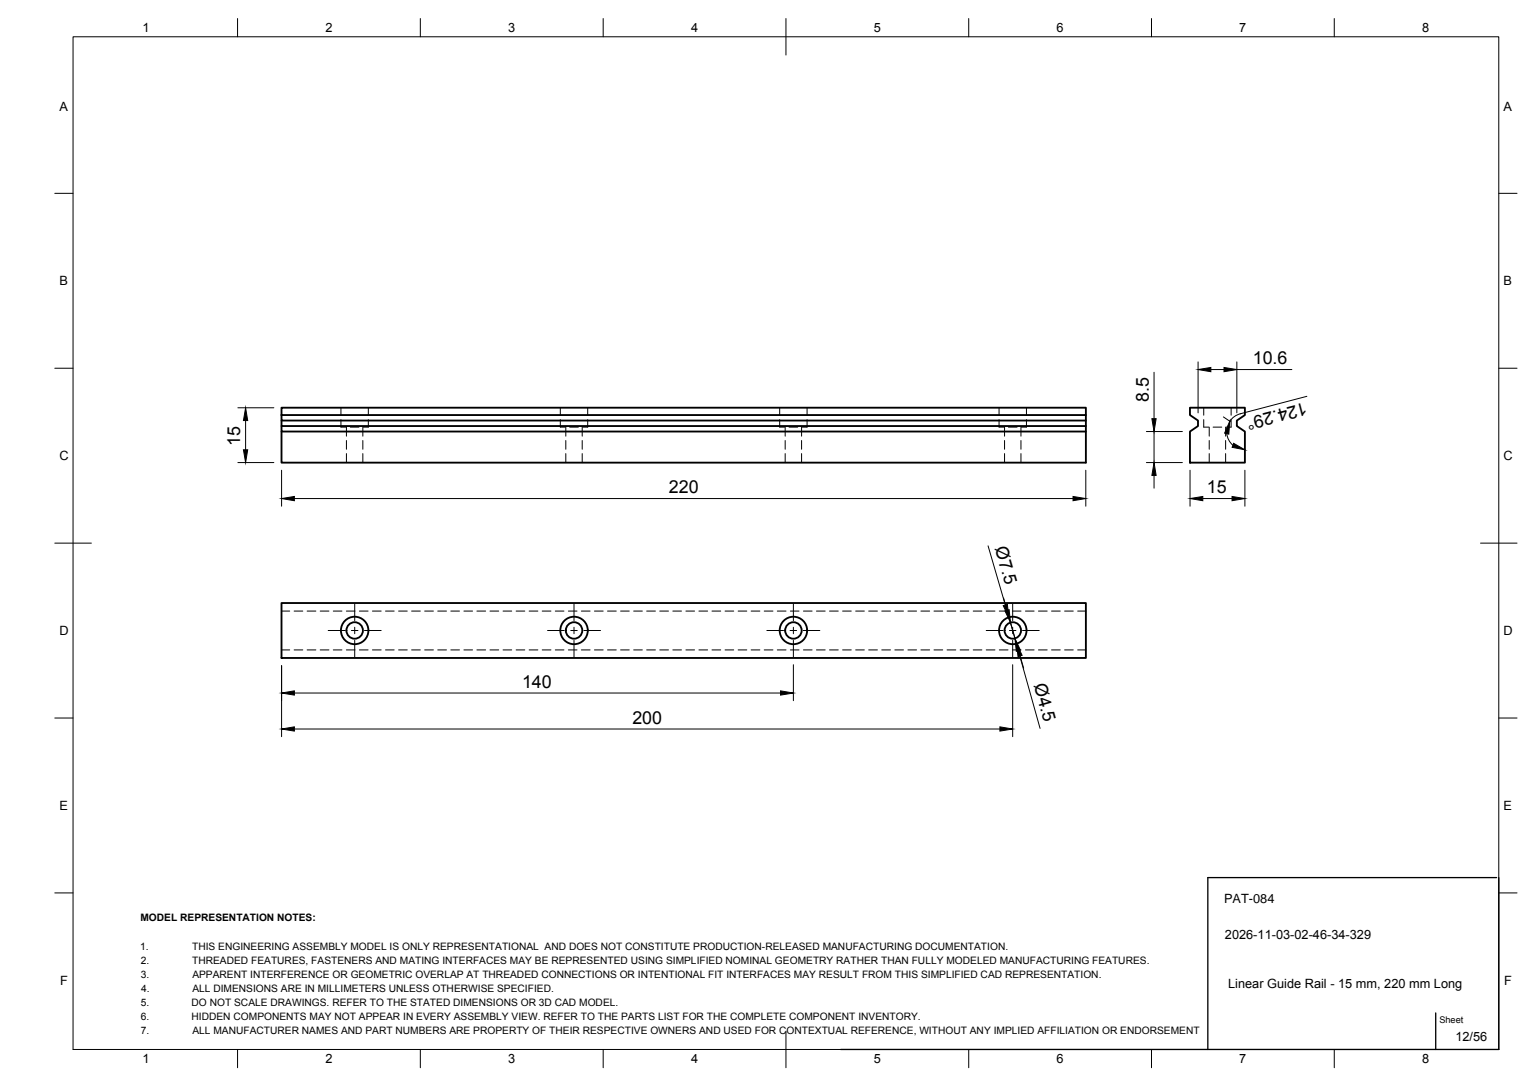
ISO-10303-21;
HEADER;
/* Generated by software containing ST-Developer
 * from STEP Tools, Inc. (www.steptools.com) 
 */

FILE_DESCRIPTION(
/* description */ ('Quick-return (Whitworth) mechanism'),
/* implementation_level */ '2;1');

FILE_NAME(
/* name */ 'Linear Guide Rail - 15 mm, 220 mm Long.step',
/* time_stamp */ '2026-10-28T03:25:57-07:00',
/* author */ (''),
/* organization */ (''),
/* preprocessor_version */ 'ST-DEVELOPER v20.2',
/* originating_system */ 'Autodesk Translation Framework v15.17.0.0',
/* authorisation */ '');

FILE_SCHEMA (('AUTOMOTIVE_DESIGN { 1 0 10303 214 3 1 1 }'));
ENDSEC;

DATA;
#10=MECHANICAL_DESIGN_GEOMETRIC_PRESENTATION_REPRESENTATION('',(#497),#14878);
#409=SHAPE_REPRESENTATION_RELATIONSHIP('SRR','None',#15077,#453);
#453=ADVANCED_BREP_SHAPE_REPRESENTATION('',(#549),#14834);
#497=STYLED_ITEM('',(#15399),#549);
#549=MANIFOLD_SOLID_BREP('Body1',#7851);
#681=FACE_BOUND('',#1729,.T.);
#682=FACE_BOUND('',#1732,.T.);
#683=FACE_BOUND('',#1735,.T.);
#684=FACE_BOUND('',#1738,.T.);
#685=FACE_BOUND('',#1748,.T.);
#686=FACE_BOUND('',#1749,.T.);
#687=FACE_BOUND('',#1750,.T.);
#688=FACE_BOUND('',#1751,.T.);
#689=FACE_BOUND('',#1758,.T.);
#690=FACE_BOUND('',#1759,.T.);
#691=FACE_BOUND('',#1760,.T.);
#692=FACE_BOUND('',#1761,.T.);
#838=PLANE('',#8669);
#839=PLANE('',#8674);
#840=PLANE('',#8679);
#841=PLANE('',#8684);
#842=PLANE('',#8694);
#843=PLANE('',#8695);
#844=PLANE('',#8696);
#845=PLANE('',#8697);
#846=PLANE('',#8698);
#847=PLANE('',#8699);
#848=PLANE('',#8700);
#849=PLANE('',#8701);
#850=PLANE('',#8702);
#851=PLANE('',#8703);
#852=PLANE('',#8704);
#853=PLANE('',#8705);
#854=PLANE('',#8706);
#855=PLANE('',#8707);
#1171=FACE_OUTER_BOUND('',#1727,.T.);
#1172=FACE_OUTER_BOUND('',#1728,.T.);
#1173=FACE_OUTER_BOUND('',#1730,.T.);
#1174=FACE_OUTER_BOUND('',#1731,.T.);
#1175=FACE_OUTER_BOUND('',#1733,.T.);
#1176=FACE_OUTER_BOUND('',#1734,.T.);
#1177=FACE_OUTER_BOUND('',#1736,.T.);
#1178=FACE_OUTER_BOUND('',#1737,.T.);
#1179=FACE_OUTER_BOUND('',#1739,.T.);
#1180=FACE_OUTER_BOUND('',#1740,.T.);
#1181=FACE_OUTER_BOUND('',#1741,.T.);
#1182=FACE_OUTER_BOUND('',#1742,.T.);
#1183=FACE_OUTER_BOUND('',#1743,.T.);
#1184=FACE_OUTER_BOUND('',#1744,.T.);
#1185=FACE_OUTER_BOUND('',#1745,.T.);
#1186=FACE_OUTER_BOUND('',#1746,.T.);
#1187=FACE_OUTER_BOUND('',#1747,.T.);
#1188=FACE_OUTER_BOUND('',#1752,.T.);
#1189=FACE_OUTER_BOUND('',#1753,.T.);
#1190=FACE_OUTER_BOUND('',#1754,.T.);
#1191=FACE_OUTER_BOUND('',#1755,.T.);
#1192=FACE_OUTER_BOUND('',#1756,.T.);
#1193=FACE_OUTER_BOUND('',#1757,.T.);
#1194=FACE_OUTER_BOUND('',#1762,.T.);
#1195=FACE_OUTER_BOUND('',#1763,.T.);
#1196=FACE_OUTER_BOUND('',#1764,.T.);
#1727=EDGE_LOOP('',(#5798,#5799,#5800,#5801));
#1728=EDGE_LOOP('',(#5802));
#1729=EDGE_LOOP('',(#5803));
#1730=EDGE_LOOP('',(#5804,#5805,#5806,#5807));
#1731=EDGE_LOOP('',(#5808));
#1732=EDGE_LOOP('',(#5809));
#1733=EDGE_LOOP('',(#5810,#5811,#5812,#5813));
#1734=EDGE_LOOP('',(#5814));
#1735=EDGE_LOOP('',(#5815));
#1736=EDGE_LOOP('',(#5816,#5817,#5818,#5819));
#1737=EDGE_LOOP('',(#5820));
#1738=EDGE_LOOP('',(#5821));
#1739=EDGE_LOOP('',(#5822,#5823,#5824,#5825));
#1740=EDGE_LOOP('',(#5826,#5827,#5828,#5829));
#1741=EDGE_LOOP('',(#5830,#5831,#5832,#5833));
#1742=EDGE_LOOP('',(#5834,#5835,#5836,#5837));
#1743=EDGE_LOOP('',(#5838,#5839,#5840,#5841));
#1744=EDGE_LOOP('',(#5842,#5843,#5844,#5845));
#1745=EDGE_LOOP('',(#5846,#5847,#5848,#5849));
#1746=EDGE_LOOP('',(#5850,#5851,#5852,#5853));
#1747=EDGE_LOOP('',(#5854,#5855,#5856,#5857));
#1748=EDGE_LOOP('',(#5858));
#1749=EDGE_LOOP('',(#5859));
#1750=EDGE_LOOP('',(#5860));
#1751=EDGE_LOOP('',(#5861));
#1752=EDGE_LOOP('',(#5862,#5863,#5864,#5865));
#1753=EDGE_LOOP('',(#5866,#5867,#5868,#5869));
#1754=EDGE_LOOP('',(#5870,#5871,#5872,#5873));
#1755=EDGE_LOOP('',(#5874,#5875,#5876,#5877));
#1756=EDGE_LOOP('',(#5878,#5879,#5880,#5881));
#1757=EDGE_LOOP('',(#5882,#5883,#5884,#5885));
#1758=EDGE_LOOP('',(#5886));
#1759=EDGE_LOOP('',(#5887));
#1760=EDGE_LOOP('',(#5888));
#1761=EDGE_LOOP('',(#5889));
#1762=EDGE_LOOP('',(#5890,#5891,#5892,#5893));
#1763=EDGE_LOOP('',(#5894,#5895,#5896,#5897,#5898,#5899,#5900,#5901,#5902,
#5903,#5904,#5905));
#1764=EDGE_LOOP('',(#5906,#5907,#5908,#5909,#5910,#5911,#5912,#5913,#5914,
#5915,#5916,#5917));
#2282=LINE('',#12668,#2805);
#2283=LINE('',#12677,#2806);
#2284=LINE('',#12686,#2807);
#2285=LINE('',#12695,#2808);
#2286=LINE('',#12703,#2809);
#2287=LINE('',#12707,#2810);
#2288=LINE('',#12711,#2811);
#2289=LINE('',#12715,#2812);
#2290=LINE('',#12719,#2813);
#2291=LINE('',#12721,#2814);
#2292=LINE('',#12723,#2815);
#2293=LINE('',#12724,#2816);
#2294=LINE('',#12727,#2817);
#2295=LINE('',#12729,#2818);
#2296=LINE('',#12730,#2819);
#2297=LINE('',#12733,#2820);
#2298=LINE('',#12735,#2821);
#2299=LINE('',#12736,#2822);
#2300=LINE('',#12739,#2823);
#2301=LINE('',#12741,#2824);
#2302=LINE('',#12742,#2825);
#2303=LINE('',#12745,#2826);
#2304=LINE('',#12747,#2827);
#2305=LINE('',#12748,#2828);
#2306=LINE('',#12751,#2829);
#2307=LINE('',#12753,#2830);
#2308=LINE('',#12754,#2831);
#2309=LINE('',#12757,#2832);
#2310=LINE('',#12759,#2833);
#2311=LINE('',#12760,#2834);
#2312=LINE('',#12763,#2835);
#2313=LINE('',#12765,#2836);
#2314=LINE('',#12766,#2837);
#2315=LINE('',#12769,#2838);
#2316=LINE('',#12771,#2839);
#2317=LINE('',#12772,#2840);
#2318=LINE('',#12775,#2841);
#2319=LINE('',#12777,#2842);
#2320=LINE('',#12778,#2843);
#2321=LINE('',#12781,#2844);
#2322=LINE('',#12783,#2845);
#2323=LINE('',#12784,#2846);
#2324=LINE('',#12786,#2847);
#2325=LINE('',#12787,#2848);
#2805=VECTOR('',#10077,0.375);
#2806=VECTOR('',#10088,0.375);
#2807=VECTOR('',#10099,0.375);
#2808=VECTOR('',#10110,0.375);
#2809=VECTOR('',#10121,0.225);
#2810=VECTOR('',#10126,0.225);
#2811=VECTOR('',#10131,0.225);
#2812=VECTOR('',#10136,0.225000000000001);
#2813=VECTOR('',#10139,1.);
#2814=VECTOR('',#10140,1.);
#2815=VECTOR('',#10141,1.);
#2816=VECTOR('',#10142,1.);
#2817=VECTOR('',#10145,1.);
#2818=VECTOR('',#10146,1.);
#2819=VECTOR('',#10147,1.);
#2820=VECTOR('',#10150,1.);
#2821=VECTOR('',#10151,1.);
#2822=VECTOR('',#10152,1.);
#2823=VECTOR('',#10155,1.);
#2824=VECTOR('',#10156,1.);
#2825=VECTOR('',#10157,1.);
#2826=VECTOR('',#10160,1.);
#2827=VECTOR('',#10161,1.);
#2828=VECTOR('',#10162,1.);
#2829=VECTOR('',#10165,1.);
#2830=VECTOR('',#10166,1.);
#2831=VECTOR('',#10167,1.);
#2832=VECTOR('',#10170,1.);
#2833=VECTOR('',#10171,1.);
#2834=VECTOR('',#10172,1.);
#2835=VECTOR('',#10175,1.);
#2836=VECTOR('',#10176,1.);
#2837=VECTOR('',#10177,1.);
#2838=VECTOR('',#10180,1.);
#2839=VECTOR('',#10181,1.);
#2840=VECTOR('',#10182,1.);
#2841=VECTOR('',#10185,1.);
#2842=VECTOR('',#10186,1.);
#2843=VECTOR('',#10187,1.);
#2844=VECTOR('',#10190,1.);
#2845=VECTOR('',#10191,1.);
#2846=VECTOR('',#10192,1.);
#2847=VECTOR('',#10195,1.);
#2848=VECTOR('',#10196,1.);
#3364=CIRCLE('',#8667,0.375);
#3365=CIRCLE('',#8668,0.375);
#3366=CIRCLE('',#8670,0.225);
#3367=CIRCLE('',#8672,0.375);
#3368=CIRCLE('',#8673,0.375);
#3369=CIRCLE('',#8675,0.225);
#3370=CIRCLE('',#8677,0.375);
#3371=CIRCLE('',#8678,0.375);
#3372=CIRCLE('',#8680,0.225);
#3373=CIRCLE('',#8682,0.375);
#3374=CIRCLE('',#8683,0.375);
#3375=CIRCLE('',#8685,0.225000000000001);
#3376=CIRCLE('',#8687,0.225);
#3377=CIRCLE('',#8689,0.225);
#3378=CIRCLE('',#8691,0.225);
#3379=CIRCLE('',#8693,0.225000000000001);
#3811=VERTEX_POINT('',#12665);
#3812=VERTEX_POINT('',#12667);
#3813=VERTEX_POINT('',#12671);
#3814=VERTEX_POINT('',#12674);
#3815=VERTEX_POINT('',#12676);
#3816=VERTEX_POINT('',#12680);
#3817=VERTEX_POINT('',#12683);
#3818=VERTEX_POINT('',#12685);
#3819=VERTEX_POINT('',#12689);
#3820=VERTEX_POINT('',#12692);
#3821=VERTEX_POINT('',#12694);
#3822=VERTEX_POINT('',#12698);
#3823=VERTEX_POINT('',#12701);
#3824=VERTEX_POINT('',#12705);
#3825=VERTEX_POINT('',#12709);
#3826=VERTEX_POINT('',#12713);
#3827=VERTEX_POINT('',#12717);
#3828=VERTEX_POINT('',#12718);
#3829=VERTEX_POINT('',#12720);
#3830=VERTEX_POINT('',#12722);
#3831=VERTEX_POINT('',#12726);
#3832=VERTEX_POINT('',#12728);
#3833=VERTEX_POINT('',#12732);
#3834=VERTEX_POINT('',#12734);
#3835=VERTEX_POINT('',#12738);
#3836=VERTEX_POINT('',#12740);
#3837=VERTEX_POINT('',#12744);
#3838=VERTEX_POINT('',#12746);
#3839=VERTEX_POINT('',#12750);
#3840=VERTEX_POINT('',#12752);
#3841=VERTEX_POINT('',#12756);
#3842=VERTEX_POINT('',#12758);
#3843=VERTEX_POINT('',#12762);
#3844=VERTEX_POINT('',#12764);
#3845=VERTEX_POINT('',#12768);
#3846=VERTEX_POINT('',#12770);
#3847=VERTEX_POINT('',#12774);
#3848=VERTEX_POINT('',#12776);
#3849=VERTEX_POINT('',#12780);
#3850=VERTEX_POINT('',#12782);
#4556=EDGE_CURVE('',#3811,#3811,#3364,.T.);
#4557=EDGE_CURVE('',#3811,#3812,#2282,.T.);
#4558=EDGE_CURVE('',#3812,#3812,#3365,.T.);
#4559=EDGE_CURVE('',#3813,#3813,#3366,.T.);
#4560=EDGE_CURVE('',#3814,#3814,#3367,.T.);
#4561=EDGE_CURVE('',#3814,#3815,#2283,.T.);
#4562=EDGE_CURVE('',#3815,#3815,#3368,.T.);
#4563=EDGE_CURVE('',#3816,#3816,#3369,.T.);
#4564=EDGE_CURVE('',#3817,#3817,#3370,.T.);
#4565=EDGE_CURVE('',#3817,#3818,#2284,.T.);
#4566=EDGE_CURVE('',#3818,#3818,#3371,.T.);
#4567=EDGE_CURVE('',#3819,#3819,#3372,.T.);
#4568=EDGE_CURVE('',#3820,#3820,#3373,.T.);
#4569=EDGE_CURVE('',#3820,#3821,#2285,.T.);
#4570=EDGE_CURVE('',#3821,#3821,#3374,.T.);
#4571=EDGE_CURVE('',#3822,#3822,#3375,.T.);
#4572=EDGE_CURVE('',#3823,#3823,#3376,.T.);
#4573=EDGE_CURVE('',#3823,#3813,#2286,.T.);
#4574=EDGE_CURVE('',#3824,#3824,#3377,.T.);
#4575=EDGE_CURVE('',#3824,#3816,#2287,.T.);
#4576=EDGE_CURVE('',#3825,#3825,#3378,.T.);
#4577=EDGE_CURVE('',#3825,#3819,#2288,.T.);
#4578=EDGE_CURVE('',#3826,#3826,#3379,.T.);
#4579=EDGE_CURVE('',#3826,#3822,#2289,.T.);
#4580=EDGE_CURVE('',#3827,#3828,#2290,.T.);
#4581=EDGE_CURVE('',#3828,#3829,#2291,.T.);
#4582=EDGE_CURVE('',#3830,#3829,#2292,.T.);
#4583=EDGE_CURVE('',#3827,#3830,#2293,.T.);
#4584=EDGE_CURVE('',#3831,#3827,#2294,.T.);
#4585=EDGE_CURVE('',#3832,#3830,#2295,.T.);
#4586=EDGE_CURVE('',#3831,#3832,#2296,.T.);
#4587=EDGE_CURVE('',#3833,#3831,#2297,.T.);
#4588=EDGE_CURVE('',#3834,#3832,#2298,.T.);
#4589=EDGE_CURVE('',#3833,#3834,#2299,.T.);
#4590=EDGE_CURVE('',#3835,#3833,#2300,.T.);
#4591=EDGE_CURVE('',#3836,#3834,#2301,.T.);
#4592=EDGE_CURVE('',#3835,#3836,#2302,.T.);
#4593=EDGE_CURVE('',#3837,#3835,#2303,.T.);
#4594=EDGE_CURVE('',#3838,#3836,#2304,.T.);
#4595=EDGE_CURVE('',#3837,#3838,#2305,.T.);
#4596=EDGE_CURVE('',#3839,#3837,#2306,.T.);
#4597=EDGE_CURVE('',#3840,#3838,#2307,.T.);
#4598=EDGE_CURVE('',#3839,#3840,#2308,.T.);
#4599=EDGE_CURVE('',#3841,#3839,#2309,.T.);
#4600=EDGE_CURVE('',#3842,#3840,#2310,.T.);
#4601=EDGE_CURVE('',#3841,#3842,#2311,.T.);
#4602=EDGE_CURVE('',#3843,#3841,#2312,.T.);
#4603=EDGE_CURVE('',#3844,#3842,#2313,.T.);
#4604=EDGE_CURVE('',#3843,#3844,#2314,.T.);
#4605=EDGE_CURVE('',#3845,#3843,#2315,.T.);
#4606=EDGE_CURVE('',#3846,#3844,#2316,.T.);
#4607=EDGE_CURVE('',#3845,#3846,#2317,.T.);
#4608=EDGE_CURVE('',#3847,#3845,#2318,.T.);
#4609=EDGE_CURVE('',#3848,#3846,#2319,.T.);
#4610=EDGE_CURVE('',#3847,#3848,#2320,.T.);
#4611=EDGE_CURVE('',#3849,#3847,#2321,.T.);
#4612=EDGE_CURVE('',#3850,#3848,#2322,.T.);
#4613=EDGE_CURVE('',#3849,#3850,#2323,.T.);
#4614=EDGE_CURVE('',#3828,#3849,#2324,.T.);
#4615=EDGE_CURVE('',#3829,#3850,#2325,.T.);
#5798=ORIENTED_EDGE('',*,*,#4556,.F.);
#5799=ORIENTED_EDGE('',*,*,#4557,.T.);
#5800=ORIENTED_EDGE('',*,*,#4558,.F.);
#5801=ORIENTED_EDGE('',*,*,#4557,.F.);
#5802=ORIENTED_EDGE('',*,*,#4556,.T.);
#5803=ORIENTED_EDGE('',*,*,#4559,.F.);
#5804=ORIENTED_EDGE('',*,*,#4560,.F.);
#5805=ORIENTED_EDGE('',*,*,#4561,.T.);
#5806=ORIENTED_EDGE('',*,*,#4562,.F.);
#5807=ORIENTED_EDGE('',*,*,#4561,.F.);
#5808=ORIENTED_EDGE('',*,*,#4560,.T.);
#5809=ORIENTED_EDGE('',*,*,#4563,.F.);
#5810=ORIENTED_EDGE('',*,*,#4564,.F.);
#5811=ORIENTED_EDGE('',*,*,#4565,.T.);
#5812=ORIENTED_EDGE('',*,*,#4566,.F.);
#5813=ORIENTED_EDGE('',*,*,#4565,.F.);
#5814=ORIENTED_EDGE('',*,*,#4564,.T.);
#5815=ORIENTED_EDGE('',*,*,#4567,.F.);
#5816=ORIENTED_EDGE('',*,*,#4568,.F.);
#5817=ORIENTED_EDGE('',*,*,#4569,.T.);
#5818=ORIENTED_EDGE('',*,*,#4570,.F.);
#5819=ORIENTED_EDGE('',*,*,#4569,.F.);
#5820=ORIENTED_EDGE('',*,*,#4568,.T.);
#5821=ORIENTED_EDGE('',*,*,#4571,.F.);
#5822=ORIENTED_EDGE('',*,*,#4572,.F.);
#5823=ORIENTED_EDGE('',*,*,#4573,.T.);
#5824=ORIENTED_EDGE('',*,*,#4559,.T.);
#5825=ORIENTED_EDGE('',*,*,#4573,.F.);
#5826=ORIENTED_EDGE('',*,*,#4574,.F.);
#5827=ORIENTED_EDGE('',*,*,#4575,.T.);
#5828=ORIENTED_EDGE('',*,*,#4563,.T.);
#5829=ORIENTED_EDGE('',*,*,#4575,.F.);
#5830=ORIENTED_EDGE('',*,*,#4576,.F.);
#5831=ORIENTED_EDGE('',*,*,#4577,.T.);
#5832=ORIENTED_EDGE('',*,*,#4567,.T.);
#5833=ORIENTED_EDGE('',*,*,#4577,.F.);
#5834=ORIENTED_EDGE('',*,*,#4578,.F.);
#5835=ORIENTED_EDGE('',*,*,#4579,.T.);
#5836=ORIENTED_EDGE('',*,*,#4571,.T.);
#5837=ORIENTED_EDGE('',*,*,#4579,.F.);
#5838=ORIENTED_EDGE('',*,*,#4580,.T.);
#5839=ORIENTED_EDGE('',*,*,#4581,.T.);
#5840=ORIENTED_EDGE('',*,*,#4582,.F.);
#5841=ORIENTED_EDGE('',*,*,#4583,.F.);
#5842=ORIENTED_EDGE('',*,*,#4584,.T.);
#5843=ORIENTED_EDGE('',*,*,#4583,.T.);
#5844=ORIENTED_EDGE('',*,*,#4585,.F.);
#5845=ORIENTED_EDGE('',*,*,#4586,.F.);
#5846=ORIENTED_EDGE('',*,*,#4587,.T.);
#5847=ORIENTED_EDGE('',*,*,#4586,.T.);
#5848=ORIENTED_EDGE('',*,*,#4588,.F.);
#5849=ORIENTED_EDGE('',*,*,#4589,.F.);
#5850=ORIENTED_EDGE('',*,*,#4590,.T.);
#5851=ORIENTED_EDGE('',*,*,#4589,.T.);
#5852=ORIENTED_EDGE('',*,*,#4591,.F.);
#5853=ORIENTED_EDGE('',*,*,#4592,.F.);
#5854=ORIENTED_EDGE('',*,*,#4593,.T.);
#5855=ORIENTED_EDGE('',*,*,#4592,.T.);
#5856=ORIENTED_EDGE('',*,*,#4594,.F.);
#5857=ORIENTED_EDGE('',*,*,#4595,.F.);
#5858=ORIENTED_EDGE('',*,*,#4570,.T.);
#5859=ORIENTED_EDGE('',*,*,#4566,.T.);
#5860=ORIENTED_EDGE('',*,*,#4562,.T.);
#5861=ORIENTED_EDGE('',*,*,#4558,.T.);
#5862=ORIENTED_EDGE('',*,*,#4596,.T.);
#5863=ORIENTED_EDGE('',*,*,#4595,.T.);
#5864=ORIENTED_EDGE('',*,*,#4597,.F.);
#5865=ORIENTED_EDGE('',*,*,#4598,.F.);
#5866=ORIENTED_EDGE('',*,*,#4599,.T.);
#5867=ORIENTED_EDGE('',*,*,#4598,.T.);
#5868=ORIENTED_EDGE('',*,*,#4600,.F.);
#5869=ORIENTED_EDGE('',*,*,#4601,.F.);
#5870=ORIENTED_EDGE('',*,*,#4602,.T.);
#5871=ORIENTED_EDGE('',*,*,#4601,.T.);
#5872=ORIENTED_EDGE('',*,*,#4603,.F.);
#5873=ORIENTED_EDGE('',*,*,#4604,.F.);
#5874=ORIENTED_EDGE('',*,*,#4605,.T.);
#5875=ORIENTED_EDGE('',*,*,#4604,.T.);
#5876=ORIENTED_EDGE('',*,*,#4606,.F.);
#5877=ORIENTED_EDGE('',*,*,#4607,.F.);
#5878=ORIENTED_EDGE('',*,*,#4608,.T.);
#5879=ORIENTED_EDGE('',*,*,#4607,.T.);
#5880=ORIENTED_EDGE('',*,*,#4609,.F.);
#5881=ORIENTED_EDGE('',*,*,#4610,.F.);
#5882=ORIENTED_EDGE('',*,*,#4611,.T.);
#5883=ORIENTED_EDGE('',*,*,#4610,.T.);
#5884=ORIENTED_EDGE('',*,*,#4612,.F.);
#5885=ORIENTED_EDGE('',*,*,#4613,.F.);
#5886=ORIENTED_EDGE('',*,*,#4572,.T.);
#5887=ORIENTED_EDGE('',*,*,#4574,.T.);
#5888=ORIENTED_EDGE('',*,*,#4576,.T.);
#5889=ORIENTED_EDGE('',*,*,#4578,.T.);
#5890=ORIENTED_EDGE('',*,*,#4614,.T.);
#5891=ORIENTED_EDGE('',*,*,#4613,.T.);
#5892=ORIENTED_EDGE('',*,*,#4615,.F.);
#5893=ORIENTED_EDGE('',*,*,#4581,.F.);
#5894=ORIENTED_EDGE('',*,*,#4615,.T.);
#5895=ORIENTED_EDGE('',*,*,#4612,.T.);
#5896=ORIENTED_EDGE('',*,*,#4609,.T.);
#5897=ORIENTED_EDGE('',*,*,#4606,.T.);
#5898=ORIENTED_EDGE('',*,*,#4603,.T.);
#5899=ORIENTED_EDGE('',*,*,#4600,.T.);
#5900=ORIENTED_EDGE('',*,*,#4597,.T.);
#5901=ORIENTED_EDGE('',*,*,#4594,.T.);
#5902=ORIENTED_EDGE('',*,*,#4591,.T.);
#5903=ORIENTED_EDGE('',*,*,#4588,.T.);
#5904=ORIENTED_EDGE('',*,*,#4585,.T.);
#5905=ORIENTED_EDGE('',*,*,#4582,.T.);
#5906=ORIENTED_EDGE('',*,*,#4614,.F.);
#5907=ORIENTED_EDGE('',*,*,#4580,.F.);
#5908=ORIENTED_EDGE('',*,*,#4584,.F.);
#5909=ORIENTED_EDGE('',*,*,#4587,.F.);
#5910=ORIENTED_EDGE('',*,*,#4590,.F.);
#5911=ORIENTED_EDGE('',*,*,#4593,.F.);
#5912=ORIENTED_EDGE('',*,*,#4596,.F.);
#5913=ORIENTED_EDGE('',*,*,#4599,.F.);
#5914=ORIENTED_EDGE('',*,*,#4602,.F.);
#5915=ORIENTED_EDGE('',*,*,#4605,.F.);
#5916=ORIENTED_EDGE('',*,*,#4608,.F.);
#5917=ORIENTED_EDGE('',*,*,#4611,.F.);
#7278=CYLINDRICAL_SURFACE('',#8666,0.375);
#7279=CYLINDRICAL_SURFACE('',#8671,0.375);
#7280=CYLINDRICAL_SURFACE('',#8676,0.375);
#7281=CYLINDRICAL_SURFACE('',#8681,0.375);
#7282=CYLINDRICAL_SURFACE('',#8686,0.225);
#7283=CYLINDRICAL_SURFACE('',#8688,0.225);
#7284=CYLINDRICAL_SURFACE('',#8690,0.225);
#7285=CYLINDRICAL_SURFACE('',#8692,0.225000000000001);
#7502=ADVANCED_FACE('',(#1171),#7278,.F.);
#7503=ADVANCED_FACE('',(#1172,#681),#838,.T.);
#7504=ADVANCED_FACE('',(#1173),#7279,.F.);
#7505=ADVANCED_FACE('',(#1174,#682),#839,.T.);
#7506=ADVANCED_FACE('',(#1175),#7280,.F.);
#7507=ADVANCED_FACE('',(#1176,#683),#840,.T.);
#7508=ADVANCED_FACE('',(#1177),#7281,.F.);
#7509=ADVANCED_FACE('',(#1178,#684),#841,.T.);
#7510=ADVANCED_FACE('',(#1179),#7282,.F.);
#7511=ADVANCED_FACE('',(#1180),#7283,.F.);
#7512=ADVANCED_FACE('',(#1181),#7284,.F.);
#7513=ADVANCED_FACE('',(#1182),#7285,.F.);
#7514=ADVANCED_FACE('',(#1183),#842,.T.);
#7515=ADVANCED_FACE('',(#1184),#843,.T.);
#7516=ADVANCED_FACE('',(#1185),#844,.T.);
#7517=ADVANCED_FACE('',(#1186),#845,.T.);
#7518=ADVANCED_FACE('',(#1187,#685,#686,#687,#688),#846,.T.);
#7519=ADVANCED_FACE('',(#1188),#847,.T.);
#7520=ADVANCED_FACE('',(#1189),#848,.T.);
#7521=ADVANCED_FACE('',(#1190),#849,.T.);
#7522=ADVANCED_FACE('',(#1191),#850,.T.);
#7523=ADVANCED_FACE('',(#1192),#851,.T.);
#7524=ADVANCED_FACE('',(#1193,#689,#690,#691,#692),#852,.T.);
#7525=ADVANCED_FACE('',(#1194),#853,.T.);
#7526=ADVANCED_FACE('',(#1195),#854,.T.);
#7527=ADVANCED_FACE('',(#1196),#855,.F.);
#7851=CLOSED_SHELL('',(#7502,#7503,#7504,#7505,#7506,#7507,#7508,#7509,
#7510,#7511,#7512,#7513,#7514,#7515,#7516,#7517,#7518,#7519,#7520,#7521,
#7522,#7523,#7524,#7525,#7526,#7527));
#8665=AXIS2_PLACEMENT_3D('',#12663,#10071,#10072);
#8666=AXIS2_PLACEMENT_3D('',#12664,#10073,#10074);
#8667=AXIS2_PLACEMENT_3D('',#12666,#10075,#10076);
#8668=AXIS2_PLACEMENT_3D('',#12669,#10078,#10079);
#8669=AXIS2_PLACEMENT_3D('',#12670,#10080,#10081);
#8670=AXIS2_PLACEMENT_3D('',#12672,#10082,#10083);
#8671=AXIS2_PLACEMENT_3D('',#12673,#10084,#10085);
#8672=AXIS2_PLACEMENT_3D('',#12675,#10086,#10087);
#8673=AXIS2_PLACEMENT_3D('',#12678,#10089,#10090);
#8674=AXIS2_PLACEMENT_3D('',#12679,#10091,#10092);
#8675=AXIS2_PLACEMENT_3D('',#12681,#10093,#10094);
#8676=AXIS2_PLACEMENT_3D('',#12682,#10095,#10096);
#8677=AXIS2_PLACEMENT_3D('',#12684,#10097,#10098);
#8678=AXIS2_PLACEMENT_3D('',#12687,#10100,#10101);
#8679=AXIS2_PLACEMENT_3D('',#12688,#10102,#10103);
#8680=AXIS2_PLACEMENT_3D('',#12690,#10104,#10105);
#8681=AXIS2_PLACEMENT_3D('',#12691,#10106,#10107);
#8682=AXIS2_PLACEMENT_3D('',#12693,#10108,#10109);
#8683=AXIS2_PLACEMENT_3D('',#12696,#10111,#10112);
#8684=AXIS2_PLACEMENT_3D('',#12697,#10113,#10114);
#8685=AXIS2_PLACEMENT_3D('',#12699,#10115,#10116);
#8686=AXIS2_PLACEMENT_3D('',#12700,#10117,#10118);
#8687=AXIS2_PLACEMENT_3D('',#12702,#10119,#10120);
#8688=AXIS2_PLACEMENT_3D('',#12704,#10122,#10123);
#8689=AXIS2_PLACEMENT_3D('',#12706,#10124,#10125);
#8690=AXIS2_PLACEMENT_3D('',#12708,#10127,#10128);
#8691=AXIS2_PLACEMENT_3D('',#12710,#10129,#10130);
#8692=AXIS2_PLACEMENT_3D('',#12712,#10132,#10133);
#8693=AXIS2_PLACEMENT_3D('',#12714,#10134,#10135);
#8694=AXIS2_PLACEMENT_3D('',#12716,#10137,#10138);
#8695=AXIS2_PLACEMENT_3D('',#12725,#10143,#10144);
#8696=AXIS2_PLACEMENT_3D('',#12731,#10148,#10149);
#8697=AXIS2_PLACEMENT_3D('',#12737,#10153,#10154);
#8698=AXIS2_PLACEMENT_3D('',#12743,#10158,#10159);
#8699=AXIS2_PLACEMENT_3D('',#12749,#10163,#10164);
#8700=AXIS2_PLACEMENT_3D('',#12755,#10168,#10169);
#8701=AXIS2_PLACEMENT_3D('',#12761,#10173,#10174);
#8702=AXIS2_PLACEMENT_3D('',#12767,#10178,#10179);
#8703=AXIS2_PLACEMENT_3D('',#12773,#10183,#10184);
#8704=AXIS2_PLACEMENT_3D('',#12779,#10188,#10189);
#8705=AXIS2_PLACEMENT_3D('',#12785,#10193,#10194);
#8706=AXIS2_PLACEMENT_3D('',#12788,#10197,#10198);
#8707=AXIS2_PLACEMENT_3D('',#12789,#10199,#10200);
#10071=DIRECTION('axis',(0.,0.,1.));
#10072=DIRECTION('refdir',(1.,0.,0.));
#10073=DIRECTION('center_axis',(0.,0.,1.));
#10074=DIRECTION('ref_axis',(1.,0.,0.));
#10075=DIRECTION('center_axis',(0.,0.,1.));
#10076=DIRECTION('ref_axis',(1.,0.,0.));
#10077=DIRECTION('',(0.,0.,1.));
#10078=DIRECTION('center_axis',(0.,0.,-1.));
#10079=DIRECTION('ref_axis',(1.,0.,0.));
#10080=DIRECTION('center_axis',(0.,0.,1.));
#10081=DIRECTION('ref_axis',(1.,0.,0.));
#10082=DIRECTION('center_axis',(0.,0.,1.));
#10083=DIRECTION('ref_axis',(1.,0.,0.));
#10084=DIRECTION('center_axis',(0.,0.,1.));
#10085=DIRECTION('ref_axis',(1.,0.,0.));
#10086=DIRECTION('center_axis',(0.,0.,1.));
#10087=DIRECTION('ref_axis',(1.,0.,0.));
#10088=DIRECTION('',(0.,0.,1.));
#10089=DIRECTION('center_axis',(0.,0.,-1.));
#10090=DIRECTION('ref_axis',(1.,0.,0.));
#10091=DIRECTION('center_axis',(0.,0.,1.));
#10092=DIRECTION('ref_axis',(1.,0.,0.));
#10093=DIRECTION('center_axis',(0.,0.,1.));
#10094=DIRECTION('ref_axis',(1.,0.,0.));
#10095=DIRECTION('center_axis',(0.,0.,1.));
#10096=DIRECTION('ref_axis',(1.,0.,0.));
#10097=DIRECTION('center_axis',(0.,0.,1.));
#10098=DIRECTION('ref_axis',(1.,0.,0.));
#10099=DIRECTION('',(0.,0.,1.));
#10100=DIRECTION('center_axis',(0.,0.,-1.));
#10101=DIRECTION('ref_axis',(1.,0.,0.));
#10102=DIRECTION('center_axis',(0.,0.,1.));
#10103=DIRECTION('ref_axis',(1.,0.,0.));
#10104=DIRECTION('center_axis',(0.,0.,1.));
#10105=DIRECTION('ref_axis',(1.,0.,0.));
#10106=DIRECTION('center_axis',(0.,0.,1.));
#10107=DIRECTION('ref_axis',(1.,0.,0.));
#10108=DIRECTION('center_axis',(0.,0.,1.));
#10109=DIRECTION('ref_axis',(1.,0.,0.));
#10110=DIRECTION('',(0.,0.,1.));
#10111=DIRECTION('center_axis',(0.,0.,-1.));
#10112=DIRECTION('ref_axis',(1.,0.,0.));
#10113=DIRECTION('center_axis',(0.,0.,1.));
#10114=DIRECTION('ref_axis',(1.,0.,0.));
#10115=DIRECTION('center_axis',(0.,0.,1.));
#10116=DIRECTION('ref_axis',(1.,0.,0.));
#10117=DIRECTION('center_axis',(0.,0.,1.));
#10118=DIRECTION('ref_axis',(1.,0.,0.));
#10119=DIRECTION('center_axis',(0.,0.,1.));
#10120=DIRECTION('ref_axis',(1.,0.,0.));
#10121=DIRECTION('',(0.,0.,1.));
#10122=DIRECTION('center_axis',(0.,0.,1.));
#10123=DIRECTION('ref_axis',(1.,0.,0.));
#10124=DIRECTION('center_axis',(0.,0.,1.));
#10125=DIRECTION('ref_axis',(1.,0.,0.));
#10126=DIRECTION('',(0.,0.,1.));
#10127=DIRECTION('center_axis',(0.,0.,1.));
#10128=DIRECTION('ref_axis',(1.,0.,0.));
#10129=DIRECTION('center_axis',(0.,0.,1.));
#10130=DIRECTION('ref_axis',(1.,0.,0.));
#10131=DIRECTION('',(0.,0.,1.));
#10132=DIRECTION('center_axis',(0.,0.,1.));
#10133=DIRECTION('ref_axis',(1.,0.,0.));
#10134=DIRECTION('center_axis',(0.,0.,1.));
#10135=DIRECTION('ref_axis',(1.,0.,0.));
#10136=DIRECTION('',(0.,0.,1.));
#10137=DIRECTION('center_axis',(0.,-0.56333682464151,0.826227342807548));
#10138=DIRECTION('ref_axis',(0.,-0.826227342807548,-0.56333682464151));
#10139=DIRECTION('',(0.,-0.826227342807548,-0.56333682464151));
#10140=DIRECTION('',(1.,0.,0.));
#10141=DIRECTION('',(0.,-0.826227342807548,-0.56333682464151));
#10142=DIRECTION('',(1.,0.,0.));
#10143=DIRECTION('center_axis',(0.,-1.,0.));
#10144=DIRECTION('ref_axis',(0.,0.,-1.));
#10145=DIRECTION('',(0.,0.,-1.));
#10146=DIRECTION('',(0.,0.,-1.));
#10147=DIRECTION('',(1.,0.,0.));
#10148=DIRECTION('center_axis',(0.,-0.56333682464151,-0.826227342807548));
#10149=DIRECTION('ref_axis',(0.,0.826227342807548,-0.56333682464151));
#10150=DIRECTION('',(0.,0.826227342807548,-0.56333682464151));
#10151=DIRECTION('',(0.,0.826227342807548,-0.56333682464151));
#10152=DIRECTION('',(1.,0.,0.));
#10153=DIRECTION('center_axis',(0.,-1.,0.));
#10154=DIRECTION('ref_axis',(0.,0.,-1.));
#10155=DIRECTION('',(0.,0.,-1.));
#10156=DIRECTION('',(0.,0.,-1.));
#10157=DIRECTION('',(1.,0.,0.));
#10158=DIRECTION('center_axis',(0.,0.,1.));
#10159=DIRECTION('ref_axis',(0.,-1.,0.));
#10160=DIRECTION('',(0.,-1.,0.));
#10161=DIRECTION('',(0.,-1.,0.));
#10162=DIRECTION('',(1.,0.,0.));
#10163=DIRECTION('center_axis',(0.,1.,0.));
#10164=DIRECTION('ref_axis',(0.,0.,1.));
#10165=DIRECTION('',(0.,0.,1.));
#10166=DIRECTION('',(0.,0.,1.));
#10167=DIRECTION('',(1.,0.,0.));
#10168=DIRECTION('center_axis',(0.,0.56333682464151,-0.826227342807548));
#10169=DIRECTION('ref_axis',(0.,0.826227342807548,0.56333682464151));
#10170=DIRECTION('',(0.,0.826227342807548,0.56333682464151));
#10171=DIRECTION('',(0.,0.826227342807548,0.56333682464151));
#10172=DIRECTION('',(1.,0.,0.));
#10173=DIRECTION('center_axis',(0.,1.,0.));
#10174=DIRECTION('ref_axis',(0.,0.,1.));
#10175=DIRECTION('',(0.,0.,1.));
#10176=DIRECTION('',(0.,0.,1.));
#10177=DIRECTION('',(1.,0.,0.));
#10178=DIRECTION('center_axis',(0.,0.56333682464151,0.826227342807548));
#10179=DIRECTION('ref_axis',(0.,-0.826227342807548,0.56333682464151));
#10180=DIRECTION('',(0.,-0.826227342807548,0.56333682464151));
#10181=DIRECTION('',(0.,-0.826227342807548,0.56333682464151));
#10182=DIRECTION('',(1.,0.,0.));
#10183=DIRECTION('center_axis',(0.,1.,0.));
#10184=DIRECTION('ref_axis',(0.,0.,1.));
#10185=DIRECTION('',(0.,0.,1.));
#10186=DIRECTION('',(0.,0.,1.));
#10187=DIRECTION('',(1.,0.,0.));
#10188=DIRECTION('center_axis',(0.,0.,-1.));
#10189=DIRECTION('ref_axis',(0.,1.,0.));
#10190=DIRECTION('',(0.,1.,0.));
#10191=DIRECTION('',(0.,1.,0.));
#10192=DIRECTION('',(1.,0.,0.));
#10193=DIRECTION('center_axis',(0.,-1.,0.));
#10194=DIRECTION('ref_axis',(0.,0.,-1.));
#10195=DIRECTION('',(0.,0.,-1.));
#10196=DIRECTION('',(0.,0.,-1.));
#10197=DIRECTION('center_axis',(1.,0.,0.));
#10198=DIRECTION('ref_axis',(0.,0.,-1.));
#10199=DIRECTION('center_axis',(1.,0.,0.));
#10200=DIRECTION('ref_axis',(0.,0.,-1.));
#12663=CARTESIAN_POINT('',(0.,0.,0.));
#12664=CARTESIAN_POINT('Origin',(14.,0.,0.97));
#12665=CARTESIAN_POINT('',(13.625,-4.59242549680257E-17,0.97));
#12666=CARTESIAN_POINT('Origin',(14.,0.,0.97));
#12667=CARTESIAN_POINT('',(13.625,4.59242549680257E-17,1.5));
#12668=CARTESIAN_POINT('',(13.625,-4.59242549680257E-17,0.97));
#12669=CARTESIAN_POINT('Origin',(14.,0.,1.5));
#12670=CARTESIAN_POINT('Origin',(14.,0.,0.97));
#12671=CARTESIAN_POINT('',(13.775,-2.75545529808154E-17,0.97));
#12672=CARTESIAN_POINT('Origin',(14.,0.,0.97));
#12673=CARTESIAN_POINT('Origin',(8.,0.,0.97));
#12674=CARTESIAN_POINT('',(7.625,-4.59242549680257E-17,0.97));
#12675=CARTESIAN_POINT('Origin',(8.,0.,0.97));
#12676=CARTESIAN_POINT('',(7.625,4.59242549680257E-17,1.5));
#12677=CARTESIAN_POINT('',(7.625,-4.59242549680257E-17,0.97));
#12678=CARTESIAN_POINT('Origin',(8.,0.,1.5));
#12679=CARTESIAN_POINT('Origin',(8.,0.,0.97));
#12680=CARTESIAN_POINT('',(7.775,-2.75545529808154E-17,0.97));
#12681=CARTESIAN_POINT('Origin',(8.,0.,0.97));
#12682=CARTESIAN_POINT('Origin',(2.,0.,0.97));
#12683=CARTESIAN_POINT('',(1.625,-4.59242549680257E-17,0.97));
#12684=CARTESIAN_POINT('Origin',(2.,0.,0.97));
#12685=CARTESIAN_POINT('',(1.625,4.59242549680257E-17,1.5));
#12686=CARTESIAN_POINT('',(1.625,-4.59242549680257E-17,0.97));
#12687=CARTESIAN_POINT('Origin',(2.,0.,1.5));
#12688=CARTESIAN_POINT('Origin',(2.,0.,0.97));
#12689=CARTESIAN_POINT('',(1.775,-2.75545529808155E-17,0.97));
#12690=CARTESIAN_POINT('Origin',(2.,0.,0.97));
#12691=CARTESIAN_POINT('Origin',(20.,0.,0.97));
#12692=CARTESIAN_POINT('',(19.625,-4.59242549680257E-17,0.97));
#12693=CARTESIAN_POINT('Origin',(20.,0.,0.97));
#12694=CARTESIAN_POINT('',(19.625,4.59242549680257E-17,1.5));
#12695=CARTESIAN_POINT('',(19.625,-4.59242549680257E-17,0.97));
#12696=CARTESIAN_POINT('Origin',(20.,0.,1.5));
#12697=CARTESIAN_POINT('Origin',(20.,0.,0.97));
#12698=CARTESIAN_POINT('',(19.775,-2.75545529808156E-17,0.97));
#12699=CARTESIAN_POINT('Origin',(20.,0.,0.97));
#12700=CARTESIAN_POINT('Origin',(14.,0.,-0.1));
#12701=CARTESIAN_POINT('',(13.775,-2.75545529808154E-17,0.));
#12702=CARTESIAN_POINT('Origin',(14.,0.,0.));
#12703=CARTESIAN_POINT('',(13.775,-2.75545529808154E-17,-0.1));
#12704=CARTESIAN_POINT('Origin',(8.,0.,-0.1));
#12705=CARTESIAN_POINT('',(7.775,-2.75545529808154E-17,0.));
#12706=CARTESIAN_POINT('Origin',(8.,0.,0.));
#12707=CARTESIAN_POINT('',(7.775,-2.75545529808154E-17,-0.1));
#12708=CARTESIAN_POINT('Origin',(2.,0.,-0.1));
#12709=CARTESIAN_POINT('',(1.775,-2.75545529808155E-17,0.));
#12710=CARTESIAN_POINT('Origin',(2.,0.,0.));
#12711=CARTESIAN_POINT('',(1.775,-2.75545529808155E-17,-0.1));
#12712=CARTESIAN_POINT('Origin',(20.,0.,-0.1));
#12713=CARTESIAN_POINT('',(19.775,-2.75545529808156E-17,0.));
#12714=CARTESIAN_POINT('Origin',(20.,0.,0.));
#12715=CARTESIAN_POINT('',(19.775,-2.75545529808156E-17,-0.1));
#12716=CARTESIAN_POINT('Origin',(0.,-0.53,1.));
#12717=CARTESIAN_POINT('',(0.,-0.53,1.));
#12718=CARTESIAN_POINT('',(0.,-0.75,0.85));
#12719=CARTESIAN_POINT('',(0.,-0.53,1.));
#12720=CARTESIAN_POINT('',(22.,-0.75,0.85));
#12721=CARTESIAN_POINT('',(0.,-0.75,0.85));
#12722=CARTESIAN_POINT('',(22.,-0.53,1.));
#12723=CARTESIAN_POINT('',(22.,-0.53,1.));
#12724=CARTESIAN_POINT('',(0.,-0.53,1.));
#12725=CARTESIAN_POINT('Origin',(0.,-0.53,1.15));
#12726=CARTESIAN_POINT('',(0.,-0.53,1.15));
#12727=CARTESIAN_POINT('',(0.,-0.53,1.15));
#12728=CARTESIAN_POINT('',(22.,-0.53,1.15));
#12729=CARTESIAN_POINT('',(22.,-0.53,1.15));
#12730=CARTESIAN_POINT('',(0.,-0.53,1.15));
#12731=CARTESIAN_POINT('Origin',(0.,-0.75,1.3));
#12732=CARTESIAN_POINT('',(0.,-0.75,1.3));
#12733=CARTESIAN_POINT('',(0.,-0.75,1.3));
#12734=CARTESIAN_POINT('',(22.,-0.75,1.3));
#12735=CARTESIAN_POINT('',(22.,-0.75,1.3));
#12736=CARTESIAN_POINT('',(0.,-0.75,1.3));
#12737=CARTESIAN_POINT('Origin',(0.,-0.75,1.5));
#12738=CARTESIAN_POINT('',(0.,-0.75,1.5));
#12739=CARTESIAN_POINT('',(0.,-0.75,1.5));
#12740=CARTESIAN_POINT('',(22.,-0.75,1.5));
#12741=CARTESIAN_POINT('',(22.,-0.75,1.5));
#12742=CARTESIAN_POINT('',(0.,-0.75,1.5));
#12743=CARTESIAN_POINT('Origin',(0.,0.75,1.5));
#12744=CARTESIAN_POINT('',(0.,0.75,1.5));
#12745=CARTESIAN_POINT('',(0.,0.75,1.5));
#12746=CARTESIAN_POINT('',(22.,0.75,1.5));
#12747=CARTESIAN_POINT('',(22.,0.75,1.5));
#12748=CARTESIAN_POINT('',(0.,0.75,1.5));
#12749=CARTESIAN_POINT('Origin',(0.,0.75,1.3));
#12750=CARTESIAN_POINT('',(0.,0.75,1.3));
#12751=CARTESIAN_POINT('',(0.,0.75,1.3));
#12752=CARTESIAN_POINT('',(22.,0.75,1.3));
#12753=CARTESIAN_POINT('',(22.,0.75,1.3));
#12754=CARTESIAN_POINT('',(0.,0.75,1.3));
#12755=CARTESIAN_POINT('Origin',(0.,0.53,1.15));
#12756=CARTESIAN_POINT('',(0.,0.53,1.15));
#12757=CARTESIAN_POINT('',(0.,0.53,1.15));
#12758=CARTESIAN_POINT('',(22.,0.53,1.15));
#12759=CARTESIAN_POINT('',(22.,0.53,1.15));
#12760=CARTESIAN_POINT('',(0.,0.53,1.15));
#12761=CARTESIAN_POINT('Origin',(0.,0.53,1.));
#12762=CARTESIAN_POINT('',(0.,0.53,1.));
#12763=CARTESIAN_POINT('',(0.,0.53,1.));
#12764=CARTESIAN_POINT('',(22.,0.53,1.));
#12765=CARTESIAN_POINT('',(22.,0.53,1.));
#12766=CARTESIAN_POINT('',(0.,0.53,1.));
#12767=CARTESIAN_POINT('Origin',(0.,0.75,0.85));
#12768=CARTESIAN_POINT('',(0.,0.75,0.85));
#12769=CARTESIAN_POINT('',(0.,0.75,0.85));
#12770=CARTESIAN_POINT('',(22.,0.75,0.85));
#12771=CARTESIAN_POINT('',(22.,0.75,0.85));
#12772=CARTESIAN_POINT('',(0.,0.75,0.85));
#12773=CARTESIAN_POINT('Origin',(0.,0.75,0.));
#12774=CARTESIAN_POINT('',(0.,0.75,0.));
#12775=CARTESIAN_POINT('',(0.,0.75,0.));
#12776=CARTESIAN_POINT('',(22.,0.75,0.));
#12777=CARTESIAN_POINT('',(22.,0.75,0.));
#12778=CARTESIAN_POINT('',(0.,0.75,0.));
#12779=CARTESIAN_POINT('Origin',(0.,-0.75,0.));
#12780=CARTESIAN_POINT('',(0.,-0.75,0.));
#12781=CARTESIAN_POINT('',(0.,-0.75,0.));
#12782=CARTESIAN_POINT('',(22.,-0.75,0.));
#12783=CARTESIAN_POINT('',(22.,-0.75,0.));
#12784=CARTESIAN_POINT('',(0.,-0.75,0.));
#12785=CARTESIAN_POINT('Origin',(0.,-0.75,0.85));
#12786=CARTESIAN_POINT('',(0.,-0.75,0.85));
#12787=CARTESIAN_POINT('',(22.,-0.75,0.85));
#12788=CARTESIAN_POINT('Origin',(22.,0.,0.75));
#12789=CARTESIAN_POINT('Origin',(0.,0.,0.75));
#14780=UNCERTAINTY_MEASURE_WITH_UNIT(LENGTH_MEASURE(0.001),#14879,
'DISTANCE_ACCURACY_VALUE',
'Maximum model space distance between geometric entities at asserted c
onnectivities');
#14824=UNCERTAINTY_MEASURE_WITH_UNIT(LENGTH_MEASURE(0.001),#14879,
'DISTANCE_ACCURACY_VALUE',
'Maximum model space distance between geometric entities at asserted c
onnectivities');
#14834=(
GEOMETRIC_REPRESENTATION_CONTEXT(3)
GLOBAL_UNCERTAINTY_ASSIGNED_CONTEXT((#14780))
GLOBAL_UNIT_ASSIGNED_CONTEXT((#14879,#14881,#14882))
REPRESENTATION_CONTEXT('','3D')
);
#14878=(
GEOMETRIC_REPRESENTATION_CONTEXT(3)
GLOBAL_UNCERTAINTY_ASSIGNED_CONTEXT((#14824))
GLOBAL_UNIT_ASSIGNED_CONTEXT((#14879,#14881,#14882))
REPRESENTATION_CONTEXT('','3D')
);
#14879=(
LENGTH_UNIT()
NAMED_UNIT(*)
SI_UNIT(.CENTI.,.METRE.)
);
#14881=(
NAMED_UNIT(*)
PLANE_ANGLE_UNIT()
SI_UNIT($,.RADIAN.)
);
#14882=(
NAMED_UNIT(*)
SI_UNIT($,.STERADIAN.)
SOLID_ANGLE_UNIT()
);
#14892=SHAPE_DEFINITION_REPRESENTATION(#14945,#15077);
#14945=PRODUCT_DEFINITION_SHAPE('',$,#15131);
#15077=SHAPE_REPRESENTATION('',(#8665),#14834);
#15121=PRODUCT_DEFINITION_CONTEXT('part definition',#15282,'design');
#15131=PRODUCT_DEFINITION('Linear Guide Rail - 15 mm, 220 mm Long',
'Linear Guide Rail - 15 mm, 220 mm Long',#15184,#15121);
#15184=PRODUCT_DEFINITION_FORMATION('',$,#15293);
#15282=APPLICATION_CONTEXT(
'Core Data for Automotive Mechanical Design Process');
#15283=PRODUCT_CONTEXT('part definition',#15282,'mechanical');
#15293=PRODUCT('Linear Guide Rail - 15 mm, 220 mm Long',
'Linear Guide Rail - 15 mm, 220 mm Long',
'Linear Guide Rail - 15 mm, 220 mm Long',(#15283));
#15393=COLOUR_RGB('Sky Blue',0.24,0.69,0.87);
#15394=FILL_AREA_STYLE_COLOUR('',#15393);
#15395=FILL_AREA_STYLE('',(#15394));
#15396=SURFACE_STYLE_FILL_AREA(#15395);
#15397=SURFACE_SIDE_STYLE('',(#15396));
#15398=SURFACE_STYLE_USAGE(.BOTH.,#15397);
#15399=PRESENTATION_STYLE_ASSIGNMENT((#15398));
ENDSEC;
END-ISO-10303-21;
